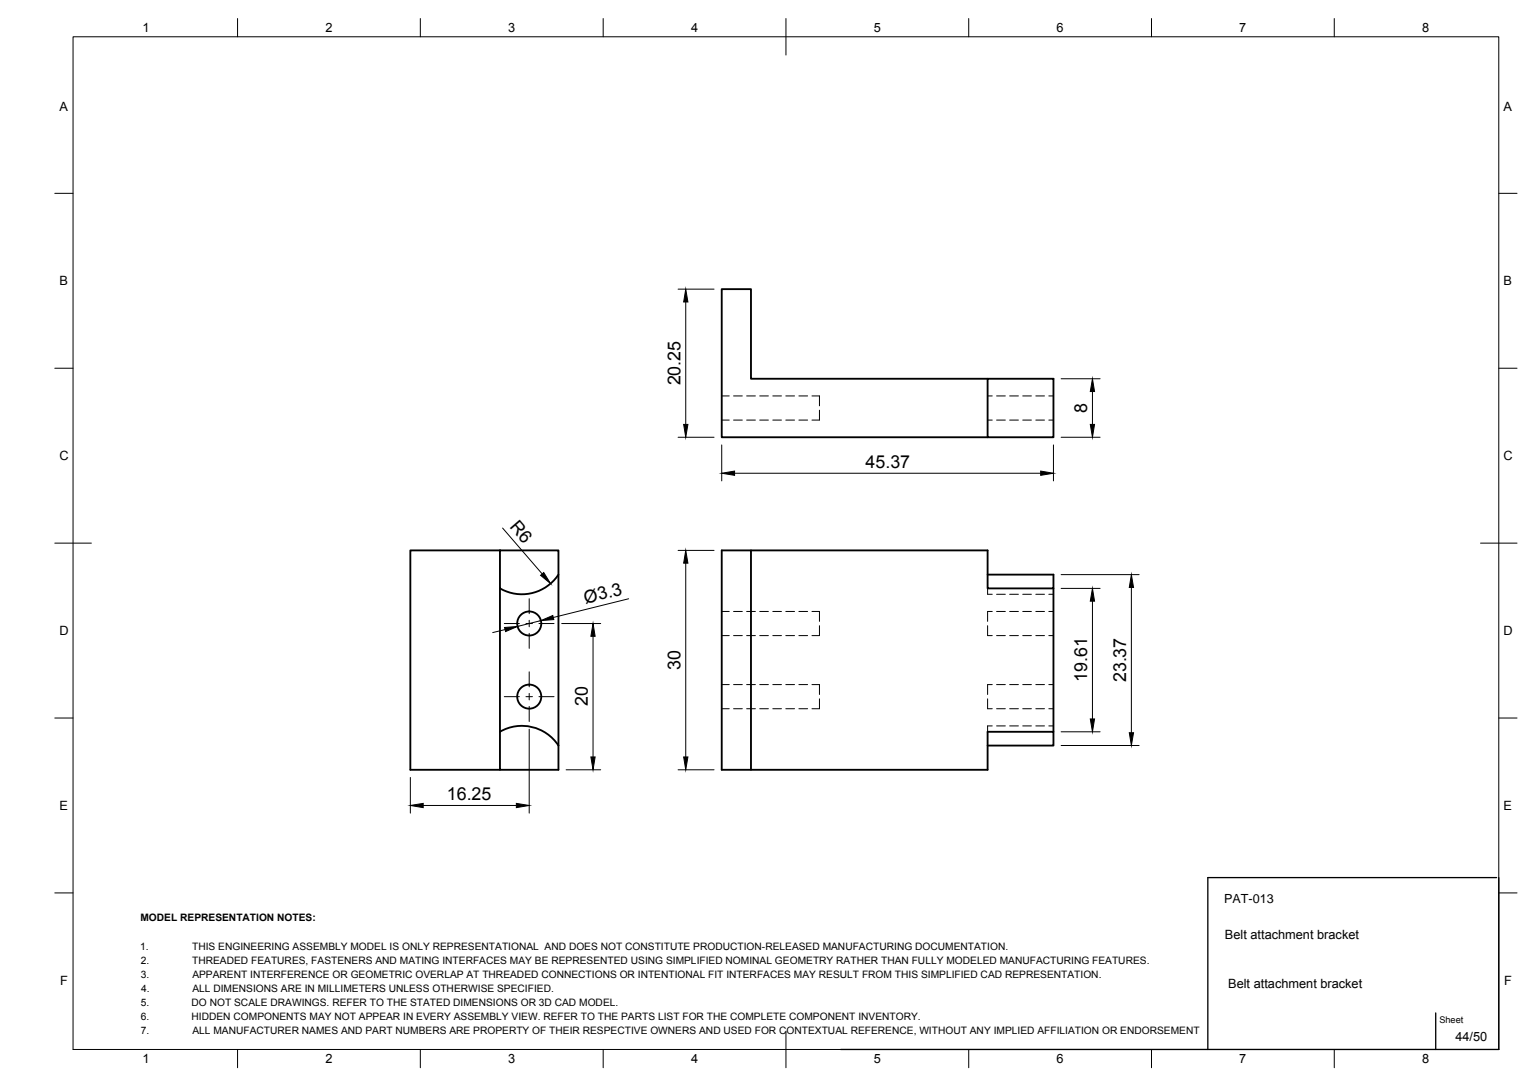
ISO-10303-21;
HEADER;
/* Generated by software containing ST-Developer
 * from STEP Tools, Inc. (www.steptools.com) 
 */

FILE_DESCRIPTION(
/* description */ ('Belt-driven linear axis on 2020 extrusion'),
/* implementation_level */ '2;1');

FILE_NAME(
/* name */ 'Belt attachment bracket.step',
/* time_stamp */ '2026-10-28T03:26:09-07:00',
/* author */ (''),
/* organization */ (''),
/* preprocessor_version */ 'ST-DEVELOPER v20.2',
/* originating_system */ 'Autodesk Translation Framework v15.17.0.0',
/* authorisation */ '');

FILE_SCHEMA (('AUTOMOTIVE_DESIGN { 1 0 10303 214 3 1 1 }'));
ENDSEC;

DATA;
#10=MECHANICAL_DESIGN_GEOMETRIC_PRESENTATION_REPRESENTATION('',(#657),#20096);
#555=SHAPE_REPRESENTATION_RELATIONSHIP('SRR','None',#20355,#601);
#601=ADVANCED_BREP_SHAPE_REPRESENTATION('',(#712),#20086);
#657=STYLED_ITEM('',(#20657),#712);
#712=MANIFOLD_SOLID_BREP('Body1',#10971);
#876=FACE_BOUND('',#2544,.T.);
#877=FACE_BOUND('',#2545,.T.);
#878=FACE_BOUND('',#2551,.T.);
#879=FACE_BOUND('',#2552,.T.);
#1157=PLANE('',#12500);
#1158=PLANE('',#12504);
#1159=PLANE('',#12505);
#1160=PLANE('',#12512);
#1161=PLANE('',#12513);
#1162=PLANE('',#12514);
#1163=PLANE('',#12518);
#1164=PLANE('',#12522);
#1165=PLANE('',#12523);
#1166=PLANE('',#12524);
#1167=PLANE('',#12525);
#1168=PLANE('',#12526);
#1169=PLANE('',#12527);
#1170=PLANE('',#12528);
#1749=FACE_OUTER_BOUND('',#2529,.T.);
#1750=FACE_OUTER_BOUND('',#2530,.T.);
#1751=FACE_OUTER_BOUND('',#2531,.T.);
#1752=FACE_OUTER_BOUND('',#2532,.T.);
#1753=FACE_OUTER_BOUND('',#2533,.T.);
#1754=FACE_OUTER_BOUND('',#2534,.T.);
#1755=FACE_OUTER_BOUND('',#2535,.T.);
#1756=FACE_OUTER_BOUND('',#2536,.T.);
#1757=FACE_OUTER_BOUND('',#2537,.T.);
#1758=FACE_OUTER_BOUND('',#2538,.T.);
#1759=FACE_OUTER_BOUND('',#2539,.T.);
#1760=FACE_OUTER_BOUND('',#2540,.T.);
#1761=FACE_OUTER_BOUND('',#2541,.T.);
#1762=FACE_OUTER_BOUND('',#2542,.T.);
#1763=FACE_OUTER_BOUND('',#2543,.T.);
#1764=FACE_OUTER_BOUND('',#2546,.T.);
#1765=FACE_OUTER_BOUND('',#2547,.T.);
#1766=FACE_OUTER_BOUND('',#2548,.T.);
#1767=FACE_OUTER_BOUND('',#2549,.T.);
#1768=FACE_OUTER_BOUND('',#2550,.T.);
#2529=EDGE_LOOP('',(#9525,#9526,#9527,#9528));
#2530=EDGE_LOOP('',(#9529));
#2531=EDGE_LOOP('',(#9530,#9531,#9532,#9533));
#2532=EDGE_LOOP('',(#9534));
#2533=EDGE_LOOP('',(#9535,#9536,#9537,#9538));
#2534=EDGE_LOOP('',(#9539,#9540,#9541,#9542));
#2535=EDGE_LOOP('',(#9543,#9544,#9545,#9546));
#2536=EDGE_LOOP('',(#9547,#9548,#9549,#9550));
#2537=EDGE_LOOP('',(#9551,#9552,#9553,#9554,#9555,#9556));
#2538=EDGE_LOOP('',(#9557,#9558,#9559,#9560,#9561,#9562,#9563,#9564));
#2539=EDGE_LOOP('',(#9565,#9566,#9567,#9568));
#2540=EDGE_LOOP('',(#9569));
#2541=EDGE_LOOP('',(#9570,#9571,#9572,#9573));
#2542=EDGE_LOOP('',(#9574));
#2543=EDGE_LOOP('',(#9575,#9576,#9577,#9578));
#2544=EDGE_LOOP('',(#9579));
#2545=EDGE_LOOP('',(#9580));
#2546=EDGE_LOOP('',(#9581,#9582,#9583,#9584));
#2547=EDGE_LOOP('',(#9585,#9586,#9587,#9588));
#2548=EDGE_LOOP('',(#9589,#9590,#9591,#9592,#9593,#9594,#9595,#9596));
#2549=EDGE_LOOP('',(#9597,#9598,#9599,#9600,#9601,#9602));
#2550=EDGE_LOOP('',(#9603,#9604,#9605,#9606));
#2551=EDGE_LOOP('',(#9607));
#2552=EDGE_LOOP('',(#9608));
#3302=LINE('',#19305,#4159);
#3303=LINE('',#19312,#4160);
#3304=LINE('',#19318,#4161);
#3305=LINE('',#19322,#4162);
#3306=LINE('',#19323,#4163);
#3307=LINE('',#19326,#4164);
#3308=LINE('',#19329,#4165);
#3309=LINE('',#19333,#4166);
#3310=LINE('',#19337,#4167);
#3311=LINE('',#19341,#4168);
#3312=LINE('',#19343,#4169);
#3313=LINE('',#19344,#4170);
#3314=LINE('',#19347,#4171);
#3315=LINE('',#19349,#4172);
#3316=LINE('',#19351,#4173);
#3317=LINE('',#19353,#4174);
#3318=LINE('',#19354,#4175);
#3319=LINE('',#19356,#4176);
#3320=LINE('',#19358,#4177);
#3321=LINE('',#19359,#4178);
#3322=LINE('',#19364,#4179);
#3323=LINE('',#19371,#4180);
#3324=LINE('',#19376,#4181);
#3325=LINE('',#19378,#4182);
#3326=LINE('',#19379,#4183);
#3327=LINE('',#19382,#4184);
#3328=LINE('',#19383,#4185);
#3329=LINE('',#19385,#4186);
#3330=LINE('',#19387,#4187);
#3331=LINE('',#19388,#4188);
#4159=VECTOR('',#15440,0.164999999999999);
#4160=VECTOR('',#15449,0.164999999999999);
#4161=VECTOR('',#15456,1.);
#4162=VECTOR('',#15459,1.);
#4163=VECTOR('',#15460,1.);
#4164=VECTOR('',#15463,1.);
#4165=VECTOR('',#15466,1.);
#4166=VECTOR('',#15469,1.);
#4167=VECTOR('',#15472,1.);
#4168=VECTOR('',#15477,1.);
#4169=VECTOR('',#15478,1.);
#4170=VECTOR('',#15479,1.);
#4171=VECTOR('',#15482,1.);
#4172=VECTOR('',#15483,1.);
#4173=VECTOR('',#15484,1.);
#4174=VECTOR('',#15485,1.);
#4175=VECTOR('',#15486,1.);
#4176=VECTOR('',#15489,1.);
#4177=VECTOR('',#15490,1.);
#4178=VECTOR('',#15491,1.);
#4179=VECTOR('',#15496,0.164999999999999);
#4180=VECTOR('',#15505,0.164999999999999);
#4181=VECTOR('',#15512,1.);
#4182=VECTOR('',#15513,1.);
#4183=VECTOR('',#15514,1.);
#4184=VECTOR('',#15517,1.);
#4185=VECTOR('',#15518,1.);
#4186=VECTOR('',#15521,1.);
#4187=VECTOR('',#15524,1.);
#4188=VECTOR('',#15525,1.);
#4836=CIRCLE('',#12498,0.164999999999999);
#4837=CIRCLE('',#12499,0.164999999999999);
#4838=CIRCLE('',#12502,0.164999999999999);
#4839=CIRCLE('',#12503,0.164999999999999);
#4840=CIRCLE('',#12506,0.6);
#4841=CIRCLE('',#12508,0.6);
#4842=CIRCLE('',#12510,0.600000000000001);
#4843=CIRCLE('',#12511,0.600000000000001);
#4844=CIRCLE('',#12516,0.164999999999999);
#4845=CIRCLE('',#12517,0.164999999999999);
#4846=CIRCLE('',#12520,0.164999999999999);
#4847=CIRCLE('',#12521,0.164999999999999);
#5661=VERTEX_POINT('',#19302);
#5662=VERTEX_POINT('',#19304);
#5663=VERTEX_POINT('',#19309);
#5664=VERTEX_POINT('',#19311);
#5665=VERTEX_POINT('',#19316);
#5666=VERTEX_POINT('',#19317);
#5667=VERTEX_POINT('',#19319);
#5668=VERTEX_POINT('',#19321);
#5669=VERTEX_POINT('',#19325);
#5670=VERTEX_POINT('',#19327);
#5671=VERTEX_POINT('',#19331);
#5672=VERTEX_POINT('',#19332);
#5673=VERTEX_POINT('',#19334);
#5674=VERTEX_POINT('',#19336);
#5675=VERTEX_POINT('',#19340);
#5676=VERTEX_POINT('',#19342);
#5677=VERTEX_POINT('',#19346);
#5678=VERTEX_POINT('',#19348);
#5679=VERTEX_POINT('',#19350);
#5680=VERTEX_POINT('',#19352);
#5681=VERTEX_POINT('',#19357);
#5682=VERTEX_POINT('',#19361);
#5683=VERTEX_POINT('',#19363);
#5684=VERTEX_POINT('',#19368);
#5685=VERTEX_POINT('',#19370);
#5686=VERTEX_POINT('',#19375);
#5687=VERTEX_POINT('',#19377);
#5688=VERTEX_POINT('',#19381);
#6977=EDGE_CURVE('',#5661,#5661,#4836,.T.);
#6978=EDGE_CURVE('',#5661,#5662,#3302,.T.);
#6979=EDGE_CURVE('',#5662,#5662,#4837,.T.);
#6980=EDGE_CURVE('',#5663,#5663,#4838,.T.);
#6981=EDGE_CURVE('',#5663,#5664,#3303,.T.);
#6982=EDGE_CURVE('',#5664,#5664,#4839,.T.);
#6983=EDGE_CURVE('',#5665,#5666,#3304,.T.);
#6984=EDGE_CURVE('',#5667,#5665,#4840,.T.);
#6985=EDGE_CURVE('',#5668,#5667,#3305,.T.);
#6986=EDGE_CURVE('',#5666,#5668,#3306,.T.);
#6987=EDGE_CURVE('',#5669,#5665,#3307,.T.);
#6988=EDGE_CURVE('',#5670,#5669,#4841,.T.);
#6989=EDGE_CURVE('',#5667,#5670,#3308,.T.);
#6990=EDGE_CURVE('',#5671,#5672,#3309,.T.);
#6991=EDGE_CURVE('',#5671,#5673,#4842,.T.);
#6992=EDGE_CURVE('',#5674,#5673,#3310,.T.);
#6993=EDGE_CURVE('',#5672,#5674,#4843,.T.);
#6994=EDGE_CURVE('',#5675,#5671,#3311,.T.);
#6995=EDGE_CURVE('',#5676,#5675,#3312,.T.);
#6996=EDGE_CURVE('',#5673,#5676,#3313,.T.);
#6997=EDGE_CURVE('',#5668,#5677,#3314,.T.);
#6998=EDGE_CURVE('',#5677,#5678,#3315,.T.);
#6999=EDGE_CURVE('',#5678,#5679,#3316,.T.);
#7000=EDGE_CURVE('',#5680,#5679,#3317,.T.);
#7001=EDGE_CURVE('',#5666,#5680,#3318,.T.);
#7002=EDGE_CURVE('',#5670,#5674,#3319,.T.);
#7003=EDGE_CURVE('',#5676,#5681,#3320,.T.);
#7004=EDGE_CURVE('',#5677,#5681,#3321,.T.);
#7005=EDGE_CURVE('',#5682,#5682,#4844,.T.);
#7006=EDGE_CURVE('',#5682,#5683,#3322,.T.);
#7007=EDGE_CURVE('',#5683,#5683,#4845,.T.);
#7008=EDGE_CURVE('',#5684,#5684,#4846,.T.);
#7009=EDGE_CURVE('',#5684,#5685,#3323,.T.);
#7010=EDGE_CURVE('',#5685,#5685,#4847,.T.);
#7011=EDGE_CURVE('',#5679,#5686,#3324,.T.);
#7012=EDGE_CURVE('',#5686,#5687,#3325,.T.);
#7013=EDGE_CURVE('',#5687,#5680,#3326,.T.);
#7014=EDGE_CURVE('',#5678,#5688,#3327,.T.);
#7015=EDGE_CURVE('',#5688,#5686,#3328,.T.);
#7016=EDGE_CURVE('',#5688,#5681,#3329,.T.);
#7017=EDGE_CURVE('',#5675,#5687,#3330,.T.);
#7018=EDGE_CURVE('',#5672,#5669,#3331,.T.);
#9525=ORIENTED_EDGE('',*,*,#6977,.F.);
#9526=ORIENTED_EDGE('',*,*,#6978,.T.);
#9527=ORIENTED_EDGE('',*,*,#6979,.T.);
#9528=ORIENTED_EDGE('',*,*,#6978,.F.);
#9529=ORIENTED_EDGE('',*,*,#6979,.F.);
#9530=ORIENTED_EDGE('',*,*,#6980,.F.);
#9531=ORIENTED_EDGE('',*,*,#6981,.T.);
#9532=ORIENTED_EDGE('',*,*,#6982,.T.);
#9533=ORIENTED_EDGE('',*,*,#6981,.F.);
#9534=ORIENTED_EDGE('',*,*,#6982,.F.);
#9535=ORIENTED_EDGE('',*,*,#6983,.F.);
#9536=ORIENTED_EDGE('',*,*,#6984,.F.);
#9537=ORIENTED_EDGE('',*,*,#6985,.F.);
#9538=ORIENTED_EDGE('',*,*,#6986,.F.);
#9539=ORIENTED_EDGE('',*,*,#6987,.F.);
#9540=ORIENTED_EDGE('',*,*,#6988,.F.);
#9541=ORIENTED_EDGE('',*,*,#6989,.F.);
#9542=ORIENTED_EDGE('',*,*,#6984,.T.);
#9543=ORIENTED_EDGE('',*,*,#6990,.F.);
#9544=ORIENTED_EDGE('',*,*,#6991,.T.);
#9545=ORIENTED_EDGE('',*,*,#6992,.F.);
#9546=ORIENTED_EDGE('',*,*,#6993,.F.);
#9547=ORIENTED_EDGE('',*,*,#6994,.F.);
#9548=ORIENTED_EDGE('',*,*,#6995,.F.);
#9549=ORIENTED_EDGE('',*,*,#6996,.F.);
#9550=ORIENTED_EDGE('',*,*,#6991,.F.);
#9551=ORIENTED_EDGE('',*,*,#6986,.T.);
#9552=ORIENTED_EDGE('',*,*,#6997,.T.);
#9553=ORIENTED_EDGE('',*,*,#6998,.T.);
#9554=ORIENTED_EDGE('',*,*,#6999,.T.);
#9555=ORIENTED_EDGE('',*,*,#7000,.F.);
#9556=ORIENTED_EDGE('',*,*,#7001,.F.);
#9557=ORIENTED_EDGE('',*,*,#6985,.T.);
#9558=ORIENTED_EDGE('',*,*,#6989,.T.);
#9559=ORIENTED_EDGE('',*,*,#7002,.T.);
#9560=ORIENTED_EDGE('',*,*,#6992,.T.);
#9561=ORIENTED_EDGE('',*,*,#6996,.T.);
#9562=ORIENTED_EDGE('',*,*,#7003,.T.);
#9563=ORIENTED_EDGE('',*,*,#7004,.F.);
#9564=ORIENTED_EDGE('',*,*,#6997,.F.);
#9565=ORIENTED_EDGE('',*,*,#7005,.F.);
#9566=ORIENTED_EDGE('',*,*,#7006,.T.);
#9567=ORIENTED_EDGE('',*,*,#7007,.F.);
#9568=ORIENTED_EDGE('',*,*,#7006,.F.);
#9569=ORIENTED_EDGE('',*,*,#7005,.T.);
#9570=ORIENTED_EDGE('',*,*,#7008,.F.);
#9571=ORIENTED_EDGE('',*,*,#7009,.T.);
#9572=ORIENTED_EDGE('',*,*,#7010,.F.);
#9573=ORIENTED_EDGE('',*,*,#7009,.F.);
#9574=ORIENTED_EDGE('',*,*,#7008,.T.);
#9575=ORIENTED_EDGE('',*,*,#7000,.T.);
#9576=ORIENTED_EDGE('',*,*,#7011,.T.);
#9577=ORIENTED_EDGE('',*,*,#7012,.T.);
#9578=ORIENTED_EDGE('',*,*,#7013,.T.);
#9579=ORIENTED_EDGE('',*,*,#7007,.T.);
#9580=ORIENTED_EDGE('',*,*,#7010,.T.);
#9581=ORIENTED_EDGE('',*,*,#7014,.T.);
#9582=ORIENTED_EDGE('',*,*,#7015,.T.);
#9583=ORIENTED_EDGE('',*,*,#7011,.F.);
#9584=ORIENTED_EDGE('',*,*,#6999,.F.);
#9585=ORIENTED_EDGE('',*,*,#7004,.T.);
#9586=ORIENTED_EDGE('',*,*,#7016,.F.);
#9587=ORIENTED_EDGE('',*,*,#7014,.F.);
#9588=ORIENTED_EDGE('',*,*,#6998,.F.);
#9589=ORIENTED_EDGE('',*,*,#6983,.T.);
#9590=ORIENTED_EDGE('',*,*,#7001,.T.);
#9591=ORIENTED_EDGE('',*,*,#7013,.F.);
#9592=ORIENTED_EDGE('',*,*,#7017,.F.);
#9593=ORIENTED_EDGE('',*,*,#6994,.T.);
#9594=ORIENTED_EDGE('',*,*,#6990,.T.);
#9595=ORIENTED_EDGE('',*,*,#7018,.T.);
#9596=ORIENTED_EDGE('',*,*,#6987,.T.);
#9597=ORIENTED_EDGE('',*,*,#6995,.T.);
#9598=ORIENTED_EDGE('',*,*,#7017,.T.);
#9599=ORIENTED_EDGE('',*,*,#7012,.F.);
#9600=ORIENTED_EDGE('',*,*,#7015,.F.);
#9601=ORIENTED_EDGE('',*,*,#7016,.T.);
#9602=ORIENTED_EDGE('',*,*,#7003,.F.);
#9603=ORIENTED_EDGE('',*,*,#6988,.T.);
#9604=ORIENTED_EDGE('',*,*,#7018,.F.);
#9605=ORIENTED_EDGE('',*,*,#6993,.T.);
#9606=ORIENTED_EDGE('',*,*,#7002,.F.);
#9607=ORIENTED_EDGE('',*,*,#6977,.T.);
#9608=ORIENTED_EDGE('',*,*,#6980,.T.);
#10283=CYLINDRICAL_SURFACE('',#12497,0.164999999999999);
#10284=CYLINDRICAL_SURFACE('',#12501,0.164999999999999);
#10285=CYLINDRICAL_SURFACE('',#12507,0.6);
#10286=CYLINDRICAL_SURFACE('',#12509,0.600000000000001);
#10287=CYLINDRICAL_SURFACE('',#12515,0.164999999999999);
#10288=CYLINDRICAL_SURFACE('',#12519,0.164999999999999);
#10800=ADVANCED_FACE('',(#1749),#10283,.F.);
#10801=ADVANCED_FACE('',(#1750),#1157,.F.);
#10802=ADVANCED_FACE('',(#1751),#10284,.F.);
#10803=ADVANCED_FACE('',(#1752),#1158,.F.);
#10804=ADVANCED_FACE('',(#1753),#1159,.F.);
#10805=ADVANCED_FACE('',(#1754),#10285,.F.);
#10806=ADVANCED_FACE('',(#1755),#10286,.F.);
#10807=ADVANCED_FACE('',(#1756),#1160,.F.);
#10808=ADVANCED_FACE('',(#1757),#1161,.T.);
#10809=ADVANCED_FACE('',(#1758),#1162,.T.);
#10810=ADVANCED_FACE('',(#1759),#10287,.F.);
#10811=ADVANCED_FACE('',(#1760),#1163,.T.);
#10812=ADVANCED_FACE('',(#1761),#10288,.F.);
#10813=ADVANCED_FACE('',(#1762),#1164,.T.);
#10814=ADVANCED_FACE('',(#1763,#876,#877),#1165,.T.);
#10815=ADVANCED_FACE('',(#1764),#1166,.T.);
#10816=ADVANCED_FACE('',(#1765),#1167,.F.);
#10817=ADVANCED_FACE('',(#1766),#1168,.T.);
#10818=ADVANCED_FACE('',(#1767),#1169,.T.);
#10819=ADVANCED_FACE('',(#1768,#878,#879),#1170,.F.);
#10971=CLOSED_SHELL('',(#10800,#10801,#10802,#10803,#10804,#10805,#10806,
#10807,#10808,#10809,#10810,#10811,#10812,#10813,#10814,#10815,#10816,#10817,
#10818,#10819));
#12496=AXIS2_PLACEMENT_3D('',#19300,#15434,#15435);
#12497=AXIS2_PLACEMENT_3D('',#19301,#15436,#15437);
#12498=AXIS2_PLACEMENT_3D('',#19303,#15438,#15439);
#12499=AXIS2_PLACEMENT_3D('',#19306,#15441,#15442);
#12500=AXIS2_PLACEMENT_3D('',#19307,#15443,#15444);
#12501=AXIS2_PLACEMENT_3D('',#19308,#15445,#15446);
#12502=AXIS2_PLACEMENT_3D('',#19310,#15447,#15448);
#12503=AXIS2_PLACEMENT_3D('',#19313,#15450,#15451);
#12504=AXIS2_PLACEMENT_3D('',#19314,#15452,#15453);
#12505=AXIS2_PLACEMENT_3D('',#19315,#15454,#15455);
#12506=AXIS2_PLACEMENT_3D('',#19320,#15457,#15458);
#12507=AXIS2_PLACEMENT_3D('',#19324,#15461,#15462);
#12508=AXIS2_PLACEMENT_3D('',#19328,#15464,#15465);
#12509=AXIS2_PLACEMENT_3D('',#19330,#15467,#15468);
#12510=AXIS2_PLACEMENT_3D('',#19335,#15470,#15471);
#12511=AXIS2_PLACEMENT_3D('',#19338,#15473,#15474);
#12512=AXIS2_PLACEMENT_3D('',#19339,#15475,#15476);
#12513=AXIS2_PLACEMENT_3D('',#19345,#15480,#15481);
#12514=AXIS2_PLACEMENT_3D('',#19355,#15487,#15488);
#12515=AXIS2_PLACEMENT_3D('',#19360,#15492,#15493);
#12516=AXIS2_PLACEMENT_3D('',#19362,#15494,#15495);
#12517=AXIS2_PLACEMENT_3D('',#19365,#15497,#15498);
#12518=AXIS2_PLACEMENT_3D('',#19366,#15499,#15500);
#12519=AXIS2_PLACEMENT_3D('',#19367,#15501,#15502);
#12520=AXIS2_PLACEMENT_3D('',#19369,#15503,#15504);
#12521=AXIS2_PLACEMENT_3D('',#19372,#15506,#15507);
#12522=AXIS2_PLACEMENT_3D('',#19373,#15508,#15509);
#12523=AXIS2_PLACEMENT_3D('',#19374,#15510,#15511);
#12524=AXIS2_PLACEMENT_3D('',#19380,#15515,#15516);
#12525=AXIS2_PLACEMENT_3D('',#19384,#15519,#15520);
#12526=AXIS2_PLACEMENT_3D('',#19386,#15522,#15523);
#12527=AXIS2_PLACEMENT_3D('',#19389,#15526,#15527);
#12528=AXIS2_PLACEMENT_3D('',#19390,#15528,#15529);
#15434=DIRECTION('axis',(0.,0.,1.));
#15435=DIRECTION('refdir',(1.,0.,0.));
#15436=DIRECTION('center_axis',(0.,0.,1.));
#15437=DIRECTION('ref_axis',(1.,0.,0.));
#15438=DIRECTION('center_axis',(0.,0.,1.));
#15439=DIRECTION('ref_axis',(1.,0.,0.));
#15440=DIRECTION('',(0.,0.,1.));
#15441=DIRECTION('center_axis',(0.,0.,1.));
#15442=DIRECTION('ref_axis',(1.,0.,0.));
#15443=DIRECTION('center_axis',(0.,0.,1.));
#15444=DIRECTION('ref_axis',(1.,0.,0.));
#15445=DIRECTION('center_axis',(0.,0.,1.));
#15446=DIRECTION('ref_axis',(1.,0.,0.));
#15447=DIRECTION('center_axis',(0.,0.,1.));
#15448=DIRECTION('ref_axis',(1.,0.,0.));
#15449=DIRECTION('',(0.,0.,1.));
#15450=DIRECTION('center_axis',(0.,0.,1.));
#15451=DIRECTION('ref_axis',(1.,0.,0.));
#15452=DIRECTION('center_axis',(0.,0.,1.));
#15453=DIRECTION('ref_axis',(1.,0.,0.));
#15454=DIRECTION('center_axis',(0.,0.,1.));
#15455=DIRECTION('ref_axis',(1.,0.,0.));
#15456=DIRECTION('',(-1.,0.,0.));
#15457=DIRECTION('center_axis',(0.,0.,1.));
#15458=DIRECTION('ref_axis',(1.,0.,0.));
#15459=DIRECTION('',(1.,0.,0.));
#15460=DIRECTION('',(0.,-1.,0.));
#15461=DIRECTION('center_axis',(0.,0.,1.));
#15462=DIRECTION('ref_axis',(1.,0.,0.));
#15463=DIRECTION('',(0.,0.,1.));
#15464=DIRECTION('center_axis',(0.,0.,1.));
#15465=DIRECTION('ref_axis',(1.,0.,0.));
#15466=DIRECTION('',(0.,0.,-1.));
#15467=DIRECTION('center_axis',(0.,0.,1.));
#15468=DIRECTION('ref_axis',(-0.973493764886257,0.228713553878167,0.));
#15469=DIRECTION('',(0.,0.,-1.));
#15470=DIRECTION('center_axis',(0.,0.,1.));
#15471=DIRECTION('ref_axis',(1.,0.,0.));
#15472=DIRECTION('',(0.,0.,1.));
#15473=DIRECTION('center_axis',(0.,0.,1.));
#15474=DIRECTION('ref_axis',(1.,0.,0.));
#15475=DIRECTION('center_axis',(0.,0.,1.));
#15476=DIRECTION('ref_axis',(1.,0.,0.));
#15477=DIRECTION('',(-1.,0.,0.));
#15478=DIRECTION('',(0.,1.,0.));
#15479=DIRECTION('',(1.,0.,0.));
#15480=DIRECTION('center_axis',(-1.,0.,0.));
#15481=DIRECTION('ref_axis',(0.,-1.,0.));
#15482=DIRECTION('',(0.,0.,1.));
#15483=DIRECTION('',(0.,-1.,0.));
#15484=DIRECTION('',(0.,0.,1.));
#15485=DIRECTION('',(0.,-1.,0.));
#15486=DIRECTION('',(0.,0.,1.));
#15487=DIRECTION('center_axis',(0.,-1.,0.));
#15488=DIRECTION('ref_axis',(1.,0.,0.));
#15489=DIRECTION('',(1.,0.,0.));
#15490=DIRECTION('',(0.,0.,1.));
#15491=DIRECTION('',(1.,0.,0.));
#15492=DIRECTION('center_axis',(0.,0.,1.));
#15493=DIRECTION('ref_axis',(1.,0.,0.));
#15494=DIRECTION('center_axis',(0.,0.,1.));
#15495=DIRECTION('ref_axis',(1.,0.,0.));
#15496=DIRECTION('',(0.,0.,1.));
#15497=DIRECTION('center_axis',(0.,0.,-1.));
#15498=DIRECTION('ref_axis',(1.,0.,0.));
#15499=DIRECTION('center_axis',(0.,0.,1.));
#15500=DIRECTION('ref_axis',(1.,0.,0.));
#15501=DIRECTION('center_axis',(0.,0.,1.));
#15502=DIRECTION('ref_axis',(1.,0.,0.));
#15503=DIRECTION('center_axis',(0.,0.,1.));
#15504=DIRECTION('ref_axis',(1.,0.,0.));
#15505=DIRECTION('',(0.,0.,1.));
#15506=DIRECTION('center_axis',(0.,0.,-1.));
#15507=DIRECTION('ref_axis',(1.,0.,0.));
#15508=DIRECTION('center_axis',(0.,0.,1.));
#15509=DIRECTION('ref_axis',(1.,0.,0.));
#15510=DIRECTION('center_axis',(0.,0.,1.));
#15511=DIRECTION('ref_axis',(1.,0.,0.));
#15512=DIRECTION('',(1.,0.,0.));
#15513=DIRECTION('',(0.,1.,0.));
#15514=DIRECTION('',(-1.,0.,0.));
#15515=DIRECTION('center_axis',(0.,-1.,0.));
#15516=DIRECTION('ref_axis',(1.,0.,0.));
#15517=DIRECTION('',(1.,0.,0.));
#15518=DIRECTION('',(0.,0.,1.));
#15519=DIRECTION('center_axis',(0.,0.,1.));
#15520=DIRECTION('ref_axis',(1.,0.,0.));
#15521=DIRECTION('',(0.,1.,0.));
#15522=DIRECTION('center_axis',(0.,1.,0.));
#15523=DIRECTION('ref_axis',(-1.,0.,0.));
#15524=DIRECTION('',(0.,0.,1.));
#15525=DIRECTION('',(-1.,0.,0.));
#15526=DIRECTION('center_axis',(1.,0.,0.));
#15527=DIRECTION('ref_axis',(0.,1.,0.));
#15528=DIRECTION('center_axis',(0.,0.,1.));
#15529=DIRECTION('ref_axis',(1.,0.,0.));
#19300=CARTESIAN_POINT('',(0.,0.,0.));
#19301=CARTESIAN_POINT('Origin',(15.5,-1.8,3.5));
#19302=CARTESIAN_POINT('',(15.335,-1.8,3.6));
#19303=CARTESIAN_POINT('Origin',(15.5,-1.8,3.6));
#19304=CARTESIAN_POINT('',(15.335,-1.8,4.5));
#19305=CARTESIAN_POINT('',(15.335,-1.8,3.5));
#19306=CARTESIAN_POINT('Origin',(15.5,-1.8,4.5));
#19307=CARTESIAN_POINT('Origin',(15.5,-1.8,4.5));
#19308=CARTESIAN_POINT('Origin',(16.5,-1.8,3.5));
#19309=CARTESIAN_POINT('',(16.335,-1.8,3.6));
#19310=CARTESIAN_POINT('Origin',(16.5,-1.8,3.6));
#19311=CARTESIAN_POINT('',(16.335,-1.8,4.5));
#19312=CARTESIAN_POINT('',(16.335,-1.8,3.5));
#19313=CARTESIAN_POINT('Origin',(16.5,-1.8,4.5));
#19314=CARTESIAN_POINT('Origin',(16.5,-1.8,4.5));
#19315=CARTESIAN_POINT('Origin',(14.5,-1.9,4.5));
#19316=CARTESIAN_POINT('',(14.8316624790355,-1.4,4.5));
#19317=CARTESIAN_POINT('',(14.5,-1.4,4.5));
#19318=CARTESIAN_POINT('',(16.,-1.4,4.5));
#19319=CARTESIAN_POINT('',(15.0196152422707,-2.2,4.5));
#19320=CARTESIAN_POINT('Origin',(14.5,-1.9,4.5));
#19321=CARTESIAN_POINT('',(14.5,-2.2,4.5));
#19322=CARTESIAN_POINT('',(14.5,-2.2,4.5));
#19323=CARTESIAN_POINT('',(14.5,-1.65,4.5));
#19324=CARTESIAN_POINT('Origin',(14.5,-1.9,3.5));
#19325=CARTESIAN_POINT('',(14.8316624790355,-1.4,3.6));
#19326=CARTESIAN_POINT('',(14.8316624790355,-1.4,3.5));
#19327=CARTESIAN_POINT('',(15.0196152422707,-2.2,3.6));
#19328=CARTESIAN_POINT('Origin',(14.5,-1.9,3.6));
#19329=CARTESIAN_POINT('',(15.0196152422707,-2.2,3.5));
#19330=CARTESIAN_POINT('Origin',(17.5,-1.9,3.5));
#19331=CARTESIAN_POINT('',(17.1683375209645,-1.4,4.5));
#19332=CARTESIAN_POINT('',(17.1683375209645,-1.4,3.6));
#19333=CARTESIAN_POINT('',(17.1683375209645,-1.4,3.5));
#19334=CARTESIAN_POINT('',(16.9803847577293,-2.2,4.5));
#19335=CARTESIAN_POINT('Origin',(17.5,-1.9,4.5));
#19336=CARTESIAN_POINT('',(16.9803847577293,-2.2,3.6));
#19337=CARTESIAN_POINT('',(16.9803847577293,-2.2,3.5));
#19338=CARTESIAN_POINT('Origin',(17.5,-1.9,3.6));
#19339=CARTESIAN_POINT('Origin',(17.5,-1.9,4.5));
#19340=CARTESIAN_POINT('',(17.5,-1.4,4.5));
#19341=CARTESIAN_POINT('',(17.5,-1.4,4.5));
#19342=CARTESIAN_POINT('',(17.5,-2.2,4.5));
#19343=CARTESIAN_POINT('',(17.5,-2.05,4.5));
#19344=CARTESIAN_POINT('',(16.,-2.2,4.5));
#19345=CARTESIAN_POINT('Origin',(14.5,-1.4,3.6));
#19346=CARTESIAN_POINT('',(14.5,-2.2,7.73661977));
#19347=CARTESIAN_POINT('',(14.5,-2.2,3.6));
#19348=CARTESIAN_POINT('',(14.5,-3.425,7.73661977));
#19349=CARTESIAN_POINT('',(14.5,-1.4,7.73661977));
#19350=CARTESIAN_POINT('',(14.5,-3.425,8.13661977));
#19351=CARTESIAN_POINT('',(14.5,-3.425,7.73661977));
#19352=CARTESIAN_POINT('',(14.5,-1.4,8.13661977));
#19353=CARTESIAN_POINT('',(14.5,-1.4,8.13661977));
#19354=CARTESIAN_POINT('',(14.5,-1.4,3.6));
#19355=CARTESIAN_POINT('Origin',(14.5,-2.2,3.6));
#19356=CARTESIAN_POINT('',(14.5,-2.2,3.6));
#19357=CARTESIAN_POINT('',(17.5,-2.2,7.73661977));
#19358=CARTESIAN_POINT('',(17.5,-2.2,3.6));
#19359=CARTESIAN_POINT('',(15.25,-2.2,7.73661977));
#19360=CARTESIAN_POINT('Origin',(15.5,-1.8,6.8));
#19361=CARTESIAN_POINT('',(15.335,-1.8,6.8));
#19362=CARTESIAN_POINT('Origin',(15.5,-1.8,6.8));
#19363=CARTESIAN_POINT('',(15.335,-1.8,8.13661977));
#19364=CARTESIAN_POINT('',(15.335,-1.8,6.8));
#19365=CARTESIAN_POINT('Origin',(15.5,-1.8,8.13661977));
#19366=CARTESIAN_POINT('Origin',(15.5,-1.8,6.8));
#19367=CARTESIAN_POINT('Origin',(16.5,-1.8,6.8));
#19368=CARTESIAN_POINT('',(16.335,-1.8,6.8));
#19369=CARTESIAN_POINT('Origin',(16.5,-1.8,6.8));
#19370=CARTESIAN_POINT('',(16.335,-1.8,8.13661977));
#19371=CARTESIAN_POINT('',(16.335,-1.8,6.8));
#19372=CARTESIAN_POINT('Origin',(16.5,-1.8,8.13661977));
#19373=CARTESIAN_POINT('Origin',(16.5,-1.8,6.8));
#19374=CARTESIAN_POINT('Origin',(16.,-2.4125,8.13661977));
#19375=CARTESIAN_POINT('',(17.5,-3.425,8.13661977));
#19376=CARTESIAN_POINT('',(14.5,-3.425,8.13661977));
#19377=CARTESIAN_POINT('',(17.5,-1.4,8.13661977));
#19378=CARTESIAN_POINT('',(17.5,-3.425,8.13661977));
#19379=CARTESIAN_POINT('',(17.5,-1.4,8.13661977));
#19380=CARTESIAN_POINT('Origin',(14.5,-3.425,7.73661977));
#19381=CARTESIAN_POINT('',(17.5,-3.425,7.73661977));
#19382=CARTESIAN_POINT('',(14.5,-3.425,7.73661977));
#19383=CARTESIAN_POINT('',(17.5,-3.425,7.73661977));
#19384=CARTESIAN_POINT('Origin',(16.,-2.4125,7.73661977));
#19385=CARTESIAN_POINT('',(17.5,-3.425,7.73661977));
#19386=CARTESIAN_POINT('Origin',(17.5,-1.4,3.6));
#19387=CARTESIAN_POINT('',(17.5,-1.4,3.6));
#19388=CARTESIAN_POINT('',(17.5,-1.4,3.6));
#19389=CARTESIAN_POINT('Origin',(17.5,-2.2,3.6));
#19390=CARTESIAN_POINT('Origin',(16.,-1.8,3.6));
#20032=UNCERTAINTY_MEASURE_WITH_UNIT(LENGTH_MEASURE(0.001),#20097,
'DISTANCE_ACCURACY_VALUE',
'Maximum model space distance between geometric entities at asserted c
onnectivities');
#20042=UNCERTAINTY_MEASURE_WITH_UNIT(LENGTH_MEASURE(0.001),#20097,
'DISTANCE_ACCURACY_VALUE',
'Maximum model space distance between geometric entities at asserted c
onnectivities');
#20086=(
GEOMETRIC_REPRESENTATION_CONTEXT(3)
GLOBAL_UNCERTAINTY_ASSIGNED_CONTEXT((#20032))
GLOBAL_UNIT_ASSIGNED_CONTEXT((#20097,#20099,#20100))
REPRESENTATION_CONTEXT('','3D')
);
#20096=(
GEOMETRIC_REPRESENTATION_CONTEXT(3)
GLOBAL_UNCERTAINTY_ASSIGNED_CONTEXT((#20042))
GLOBAL_UNIT_ASSIGNED_CONTEXT((#20097,#20099,#20100))
REPRESENTATION_CONTEXT('','3D')
);
#20097=(
LENGTH_UNIT()
NAMED_UNIT(*)
SI_UNIT(.CENTI.,.METRE.)
);
#20099=(
NAMED_UNIT(*)
PLANE_ANGLE_UNIT()
SI_UNIT($,.RADIAN.)
);
#20100=(
NAMED_UNIT(*)
SI_UNIT($,.STERADIAN.)
SOLID_ANGLE_UNIT()
);
#20144=SHAPE_DEFINITION_REPRESENTATION(#20202,#20355);
#20202=PRODUCT_DEFINITION_SHAPE('',$,#20409);
#20355=SHAPE_REPRESENTATION('',(#12496),#20086);
#20365=PRODUCT_DEFINITION_CONTEXT('part definition',#20526,'design');
#20409=PRODUCT_DEFINITION('Belt attachment bracket',
'Belt attachment bracket',#20462,#20365);
#20462=PRODUCT_DEFINITION_FORMATION('',$,#20571);
#20526=APPLICATION_CONTEXT(
'Core Data for Automotive Mechanical Design Process');
#20527=PRODUCT_CONTEXT('part definition',#20526,'mechanical');
#20571=PRODUCT('Belt attachment bracket','Belt attachment bracket',
'Belt attachment bracket',(#20527));
#20651=COLOUR_RGB('Black',0.12,0.14,0.17);
#20652=FILL_AREA_STYLE_COLOUR('',#20651);
#20653=FILL_AREA_STYLE('',(#20652));
#20654=SURFACE_STYLE_FILL_AREA(#20653);
#20655=SURFACE_SIDE_STYLE('',(#20654));
#20656=SURFACE_STYLE_USAGE(.BOTH.,#20655);
#20657=PRESENTATION_STYLE_ASSIGNMENT((#20656));
ENDSEC;
END-ISO-10303-21;
